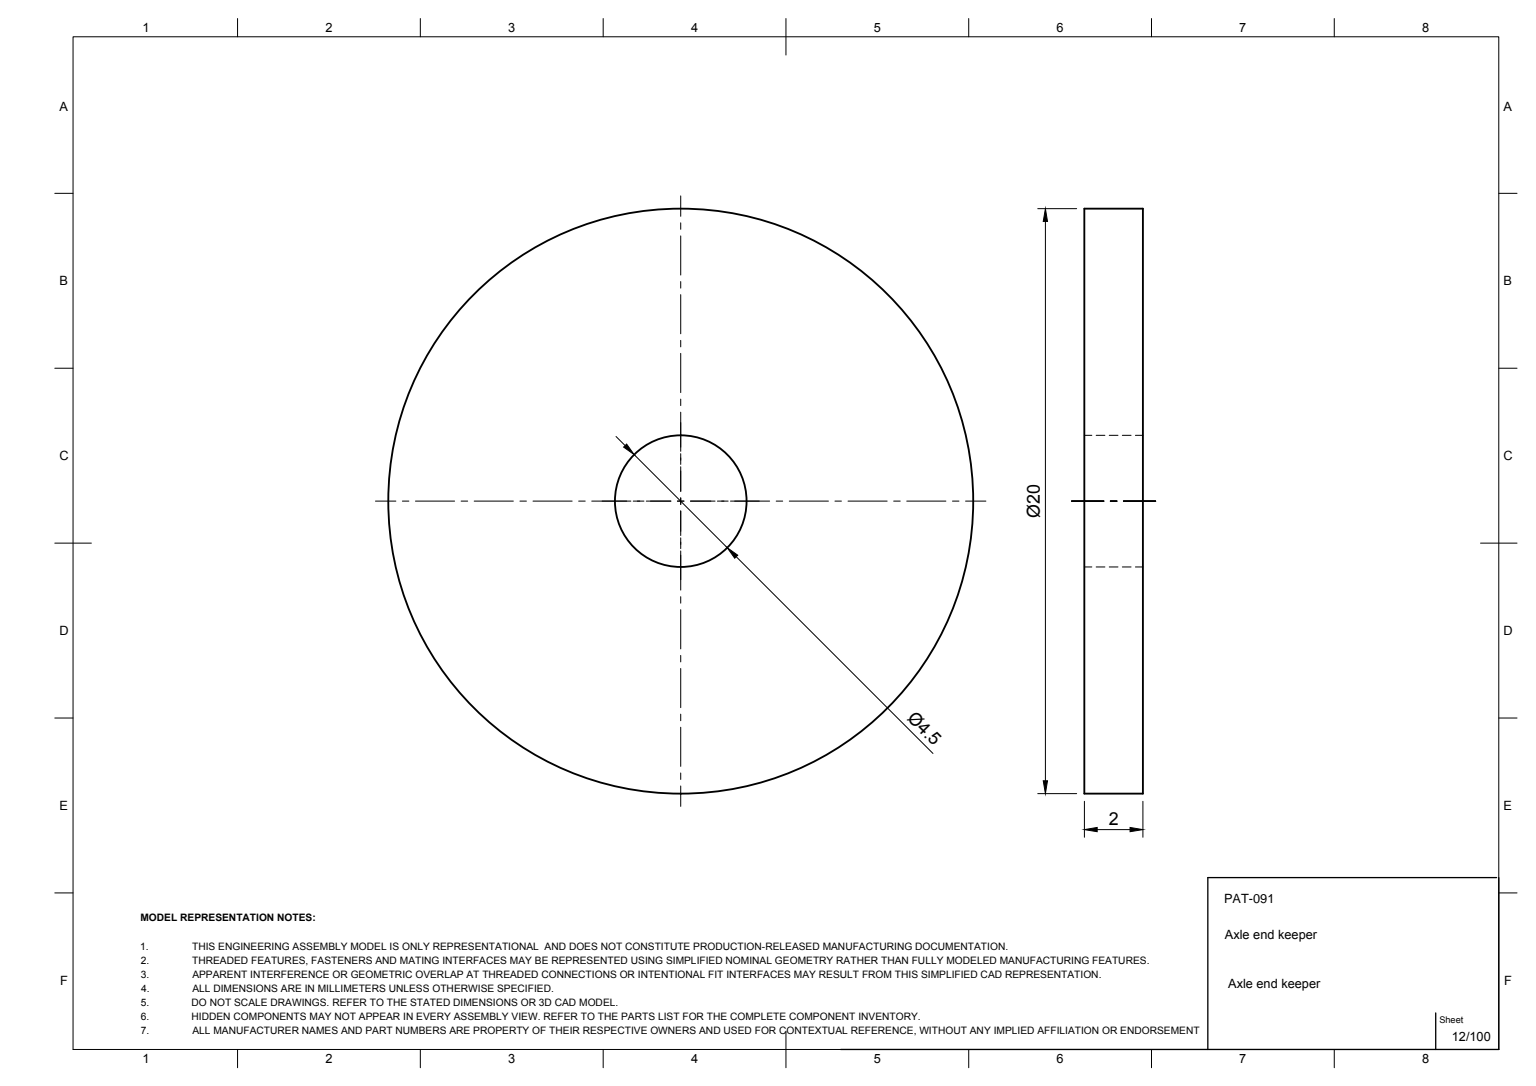
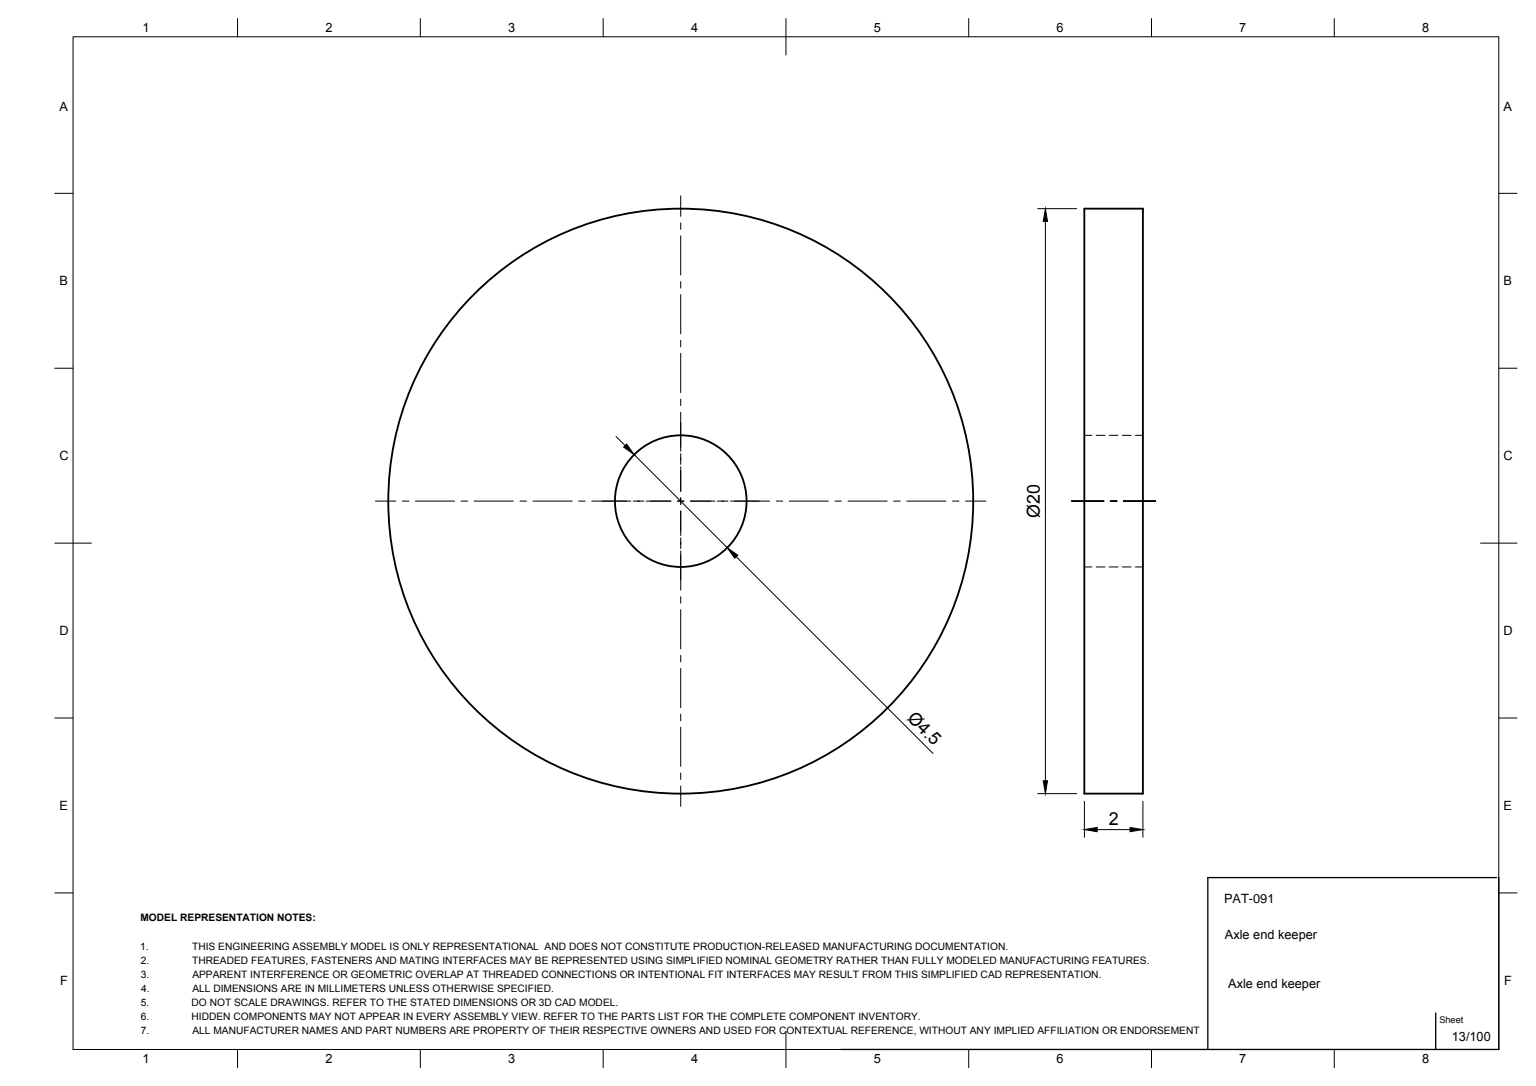
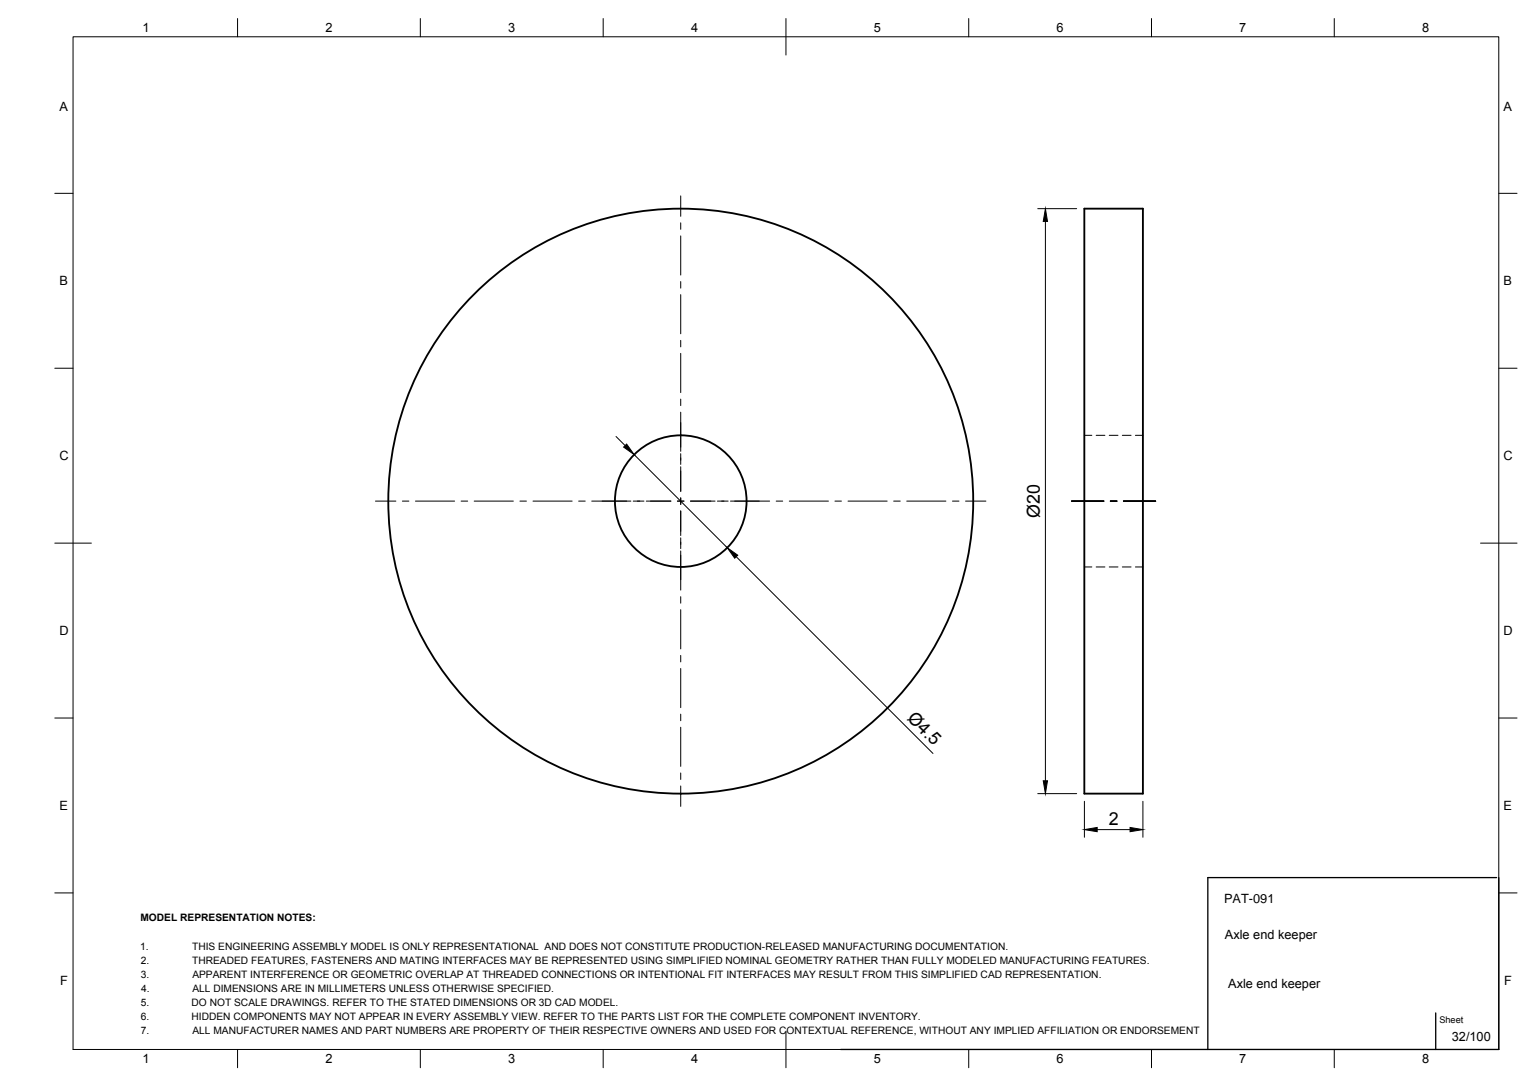
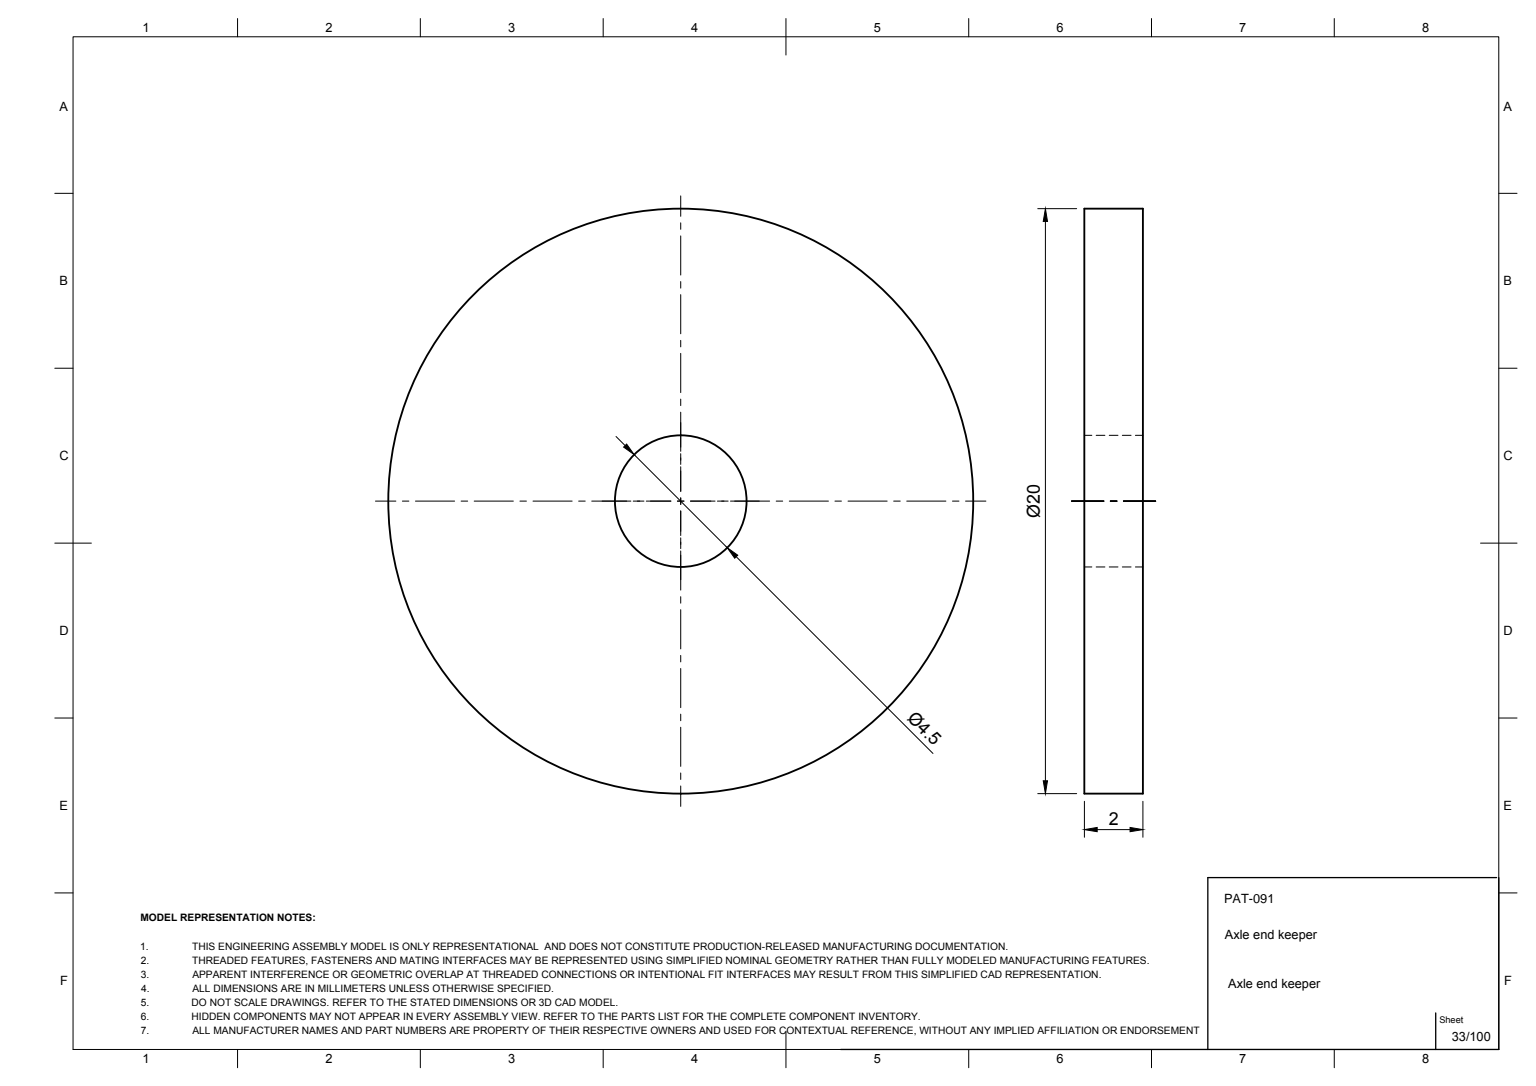
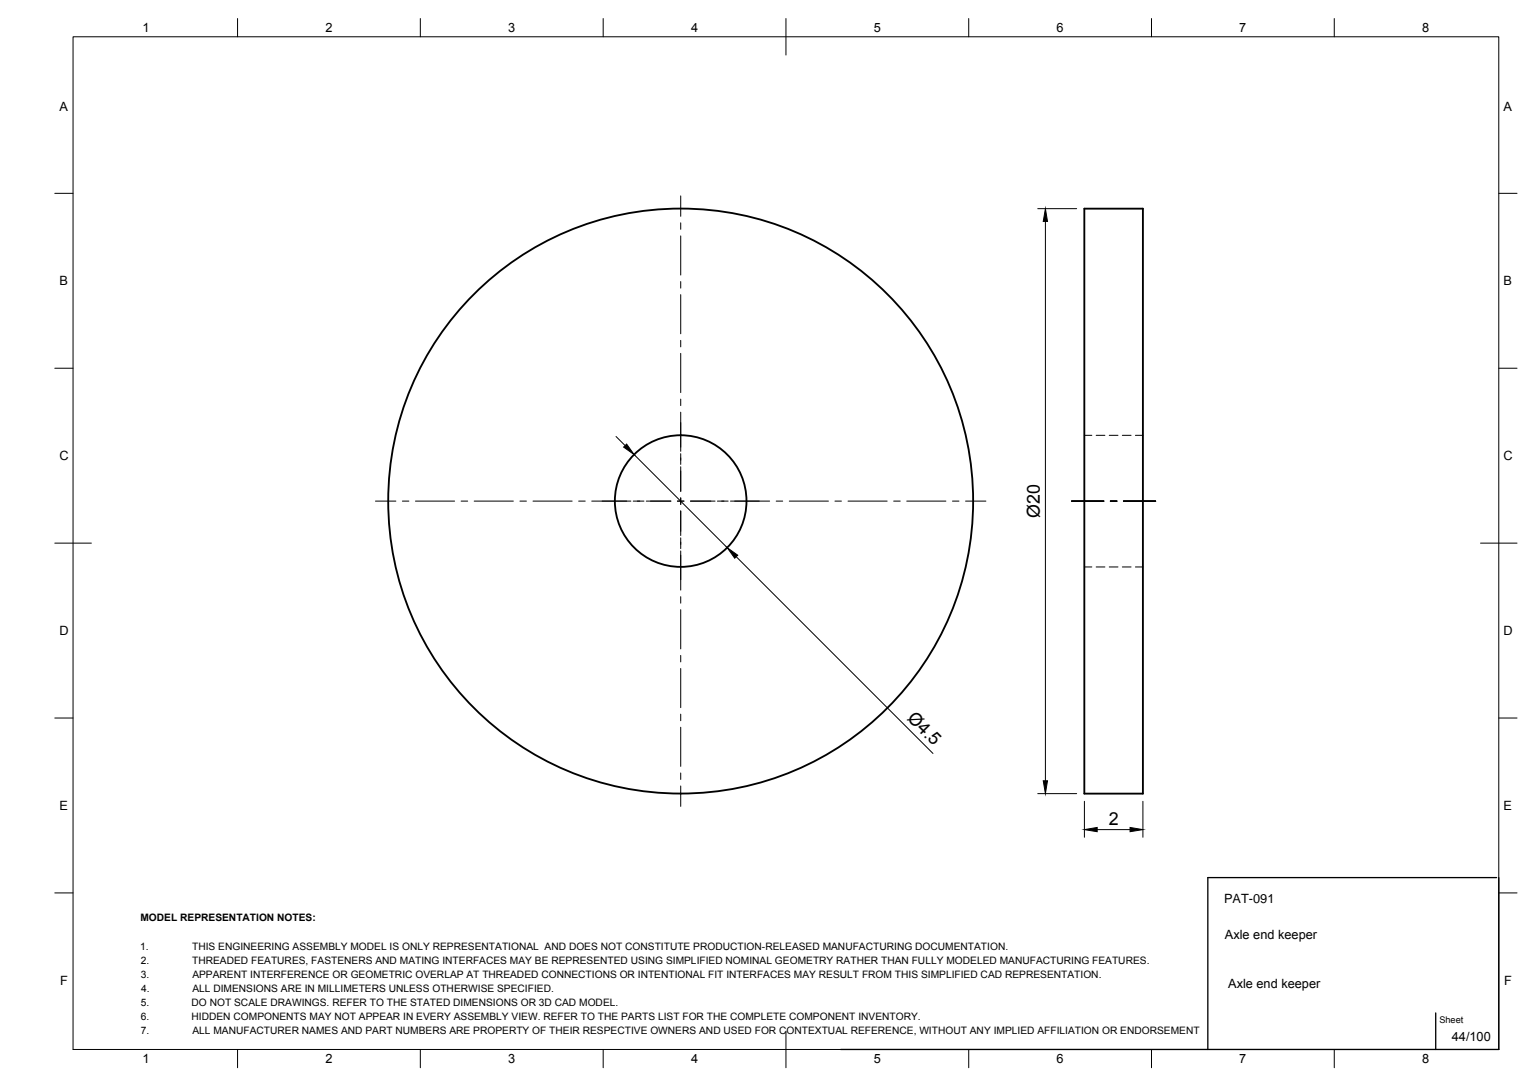
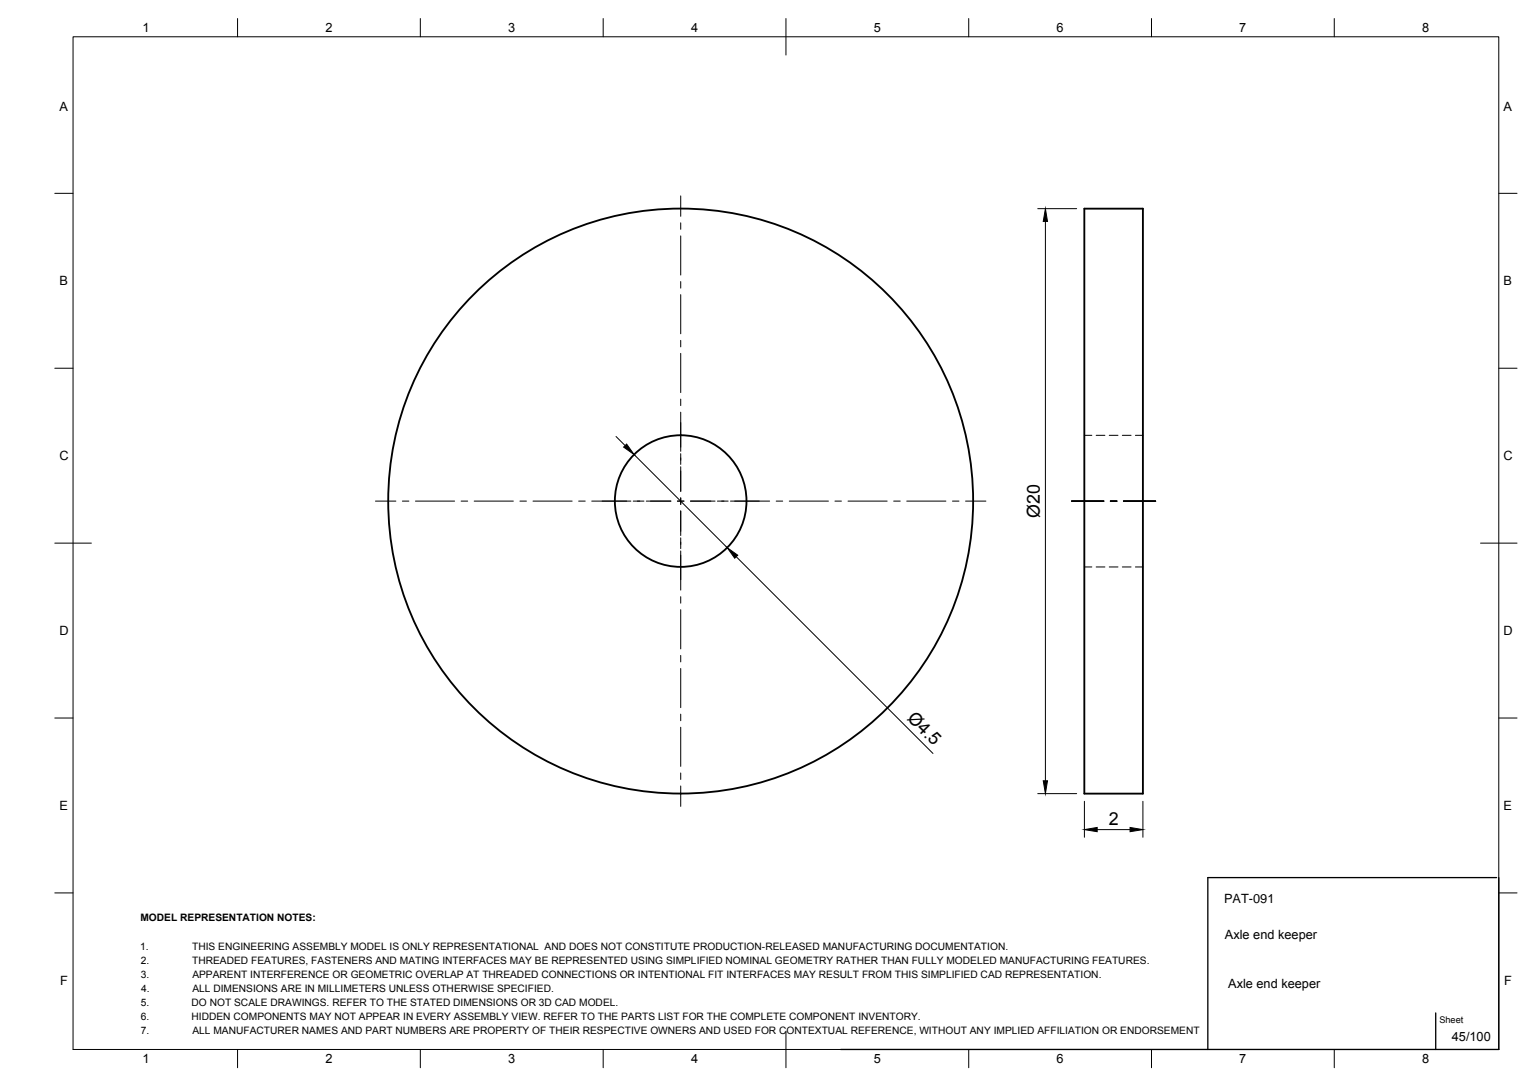
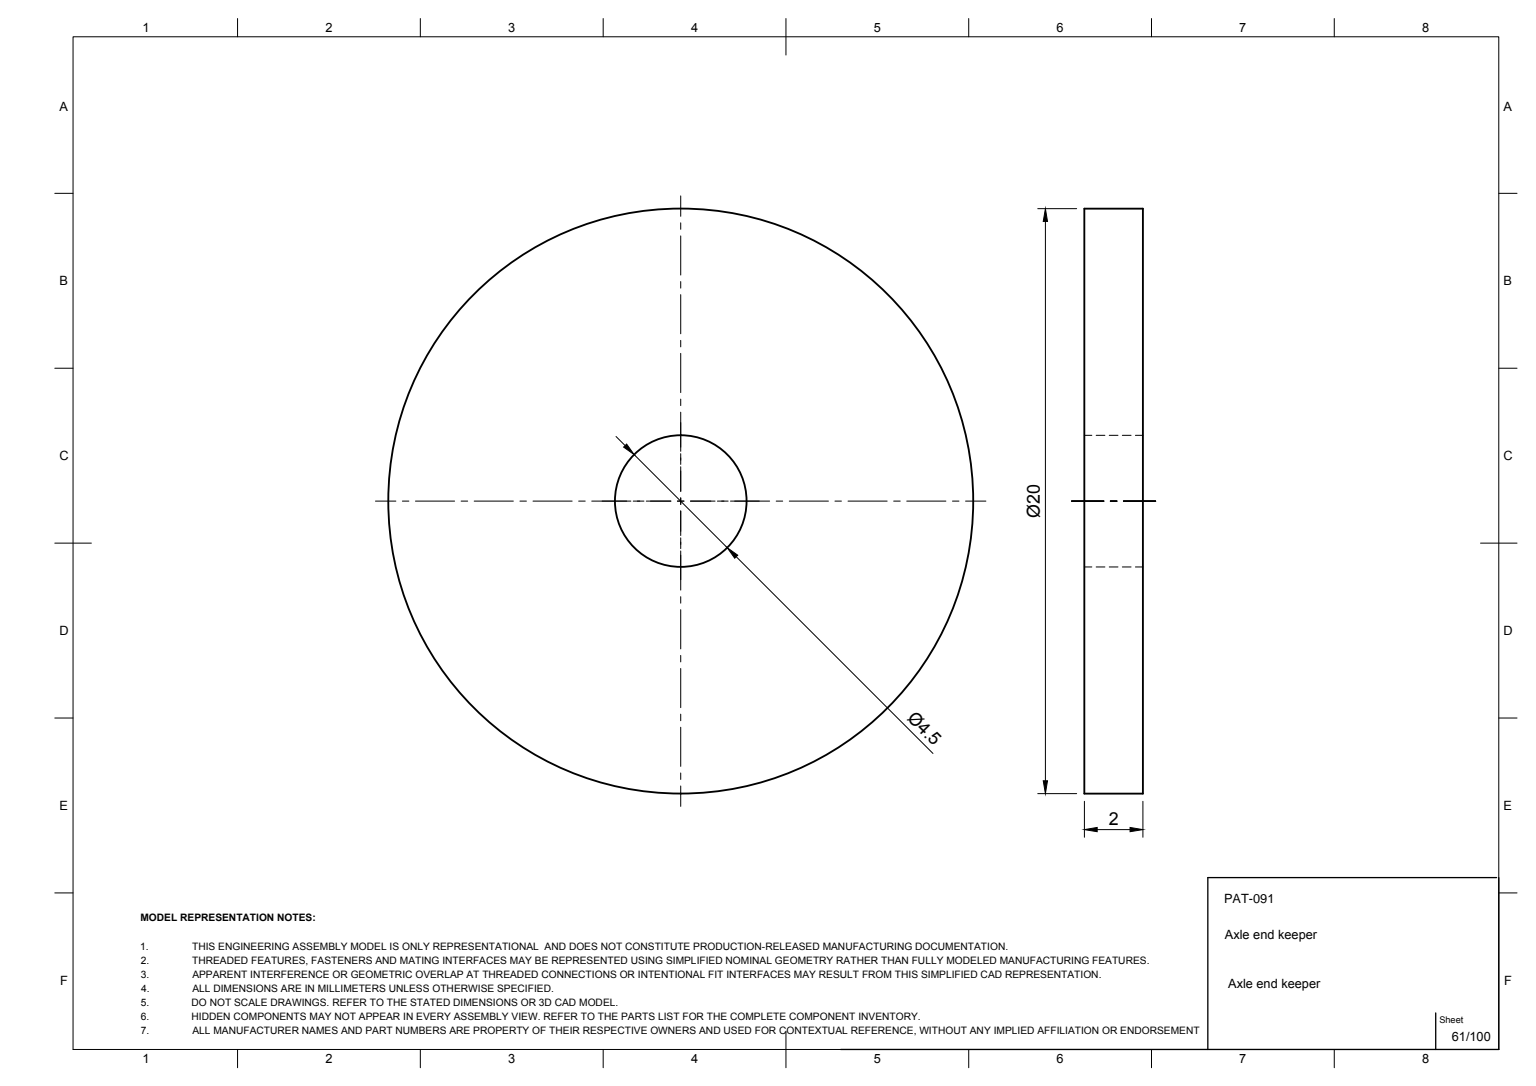
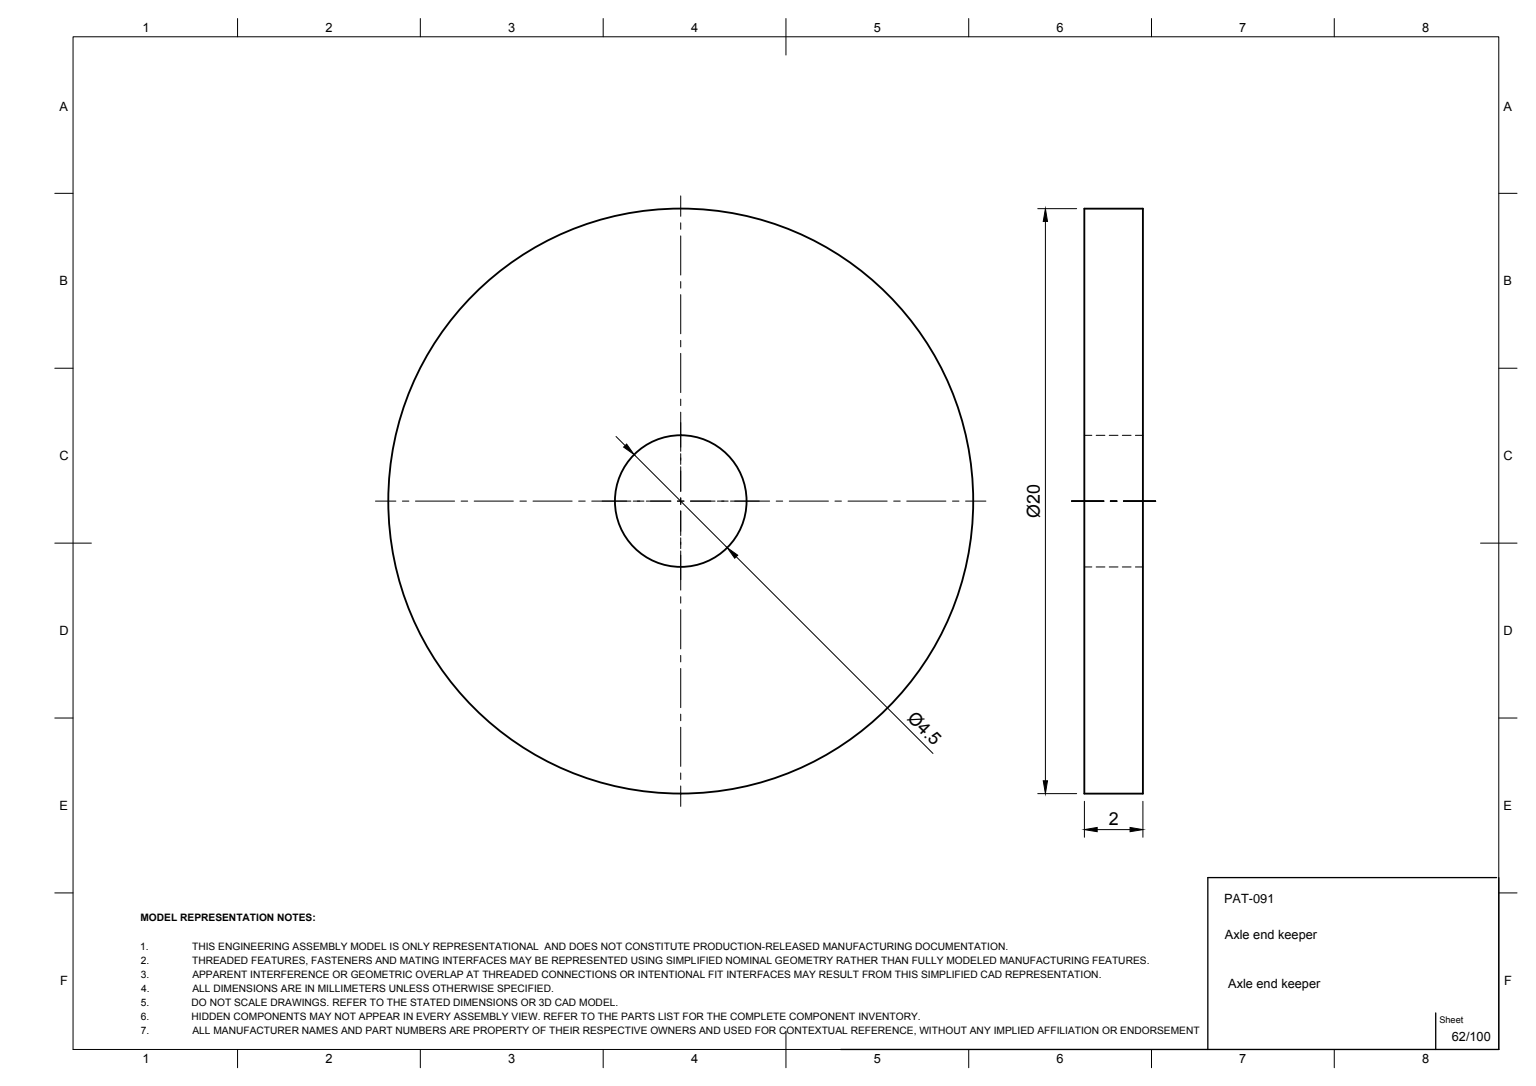
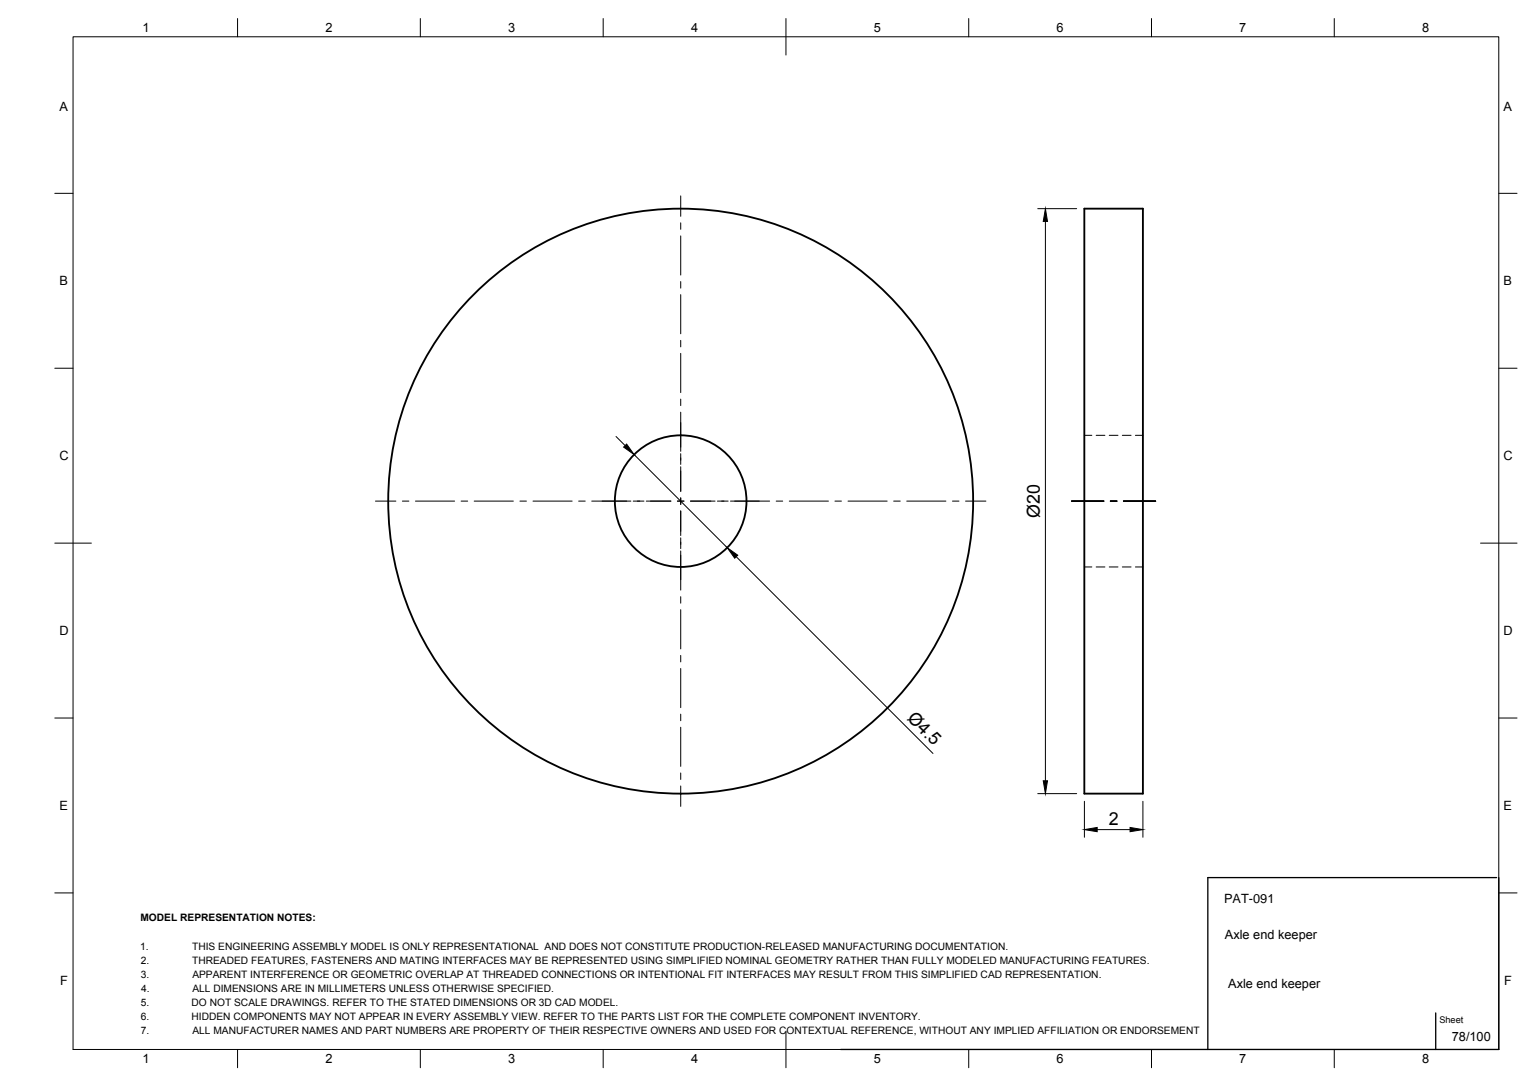
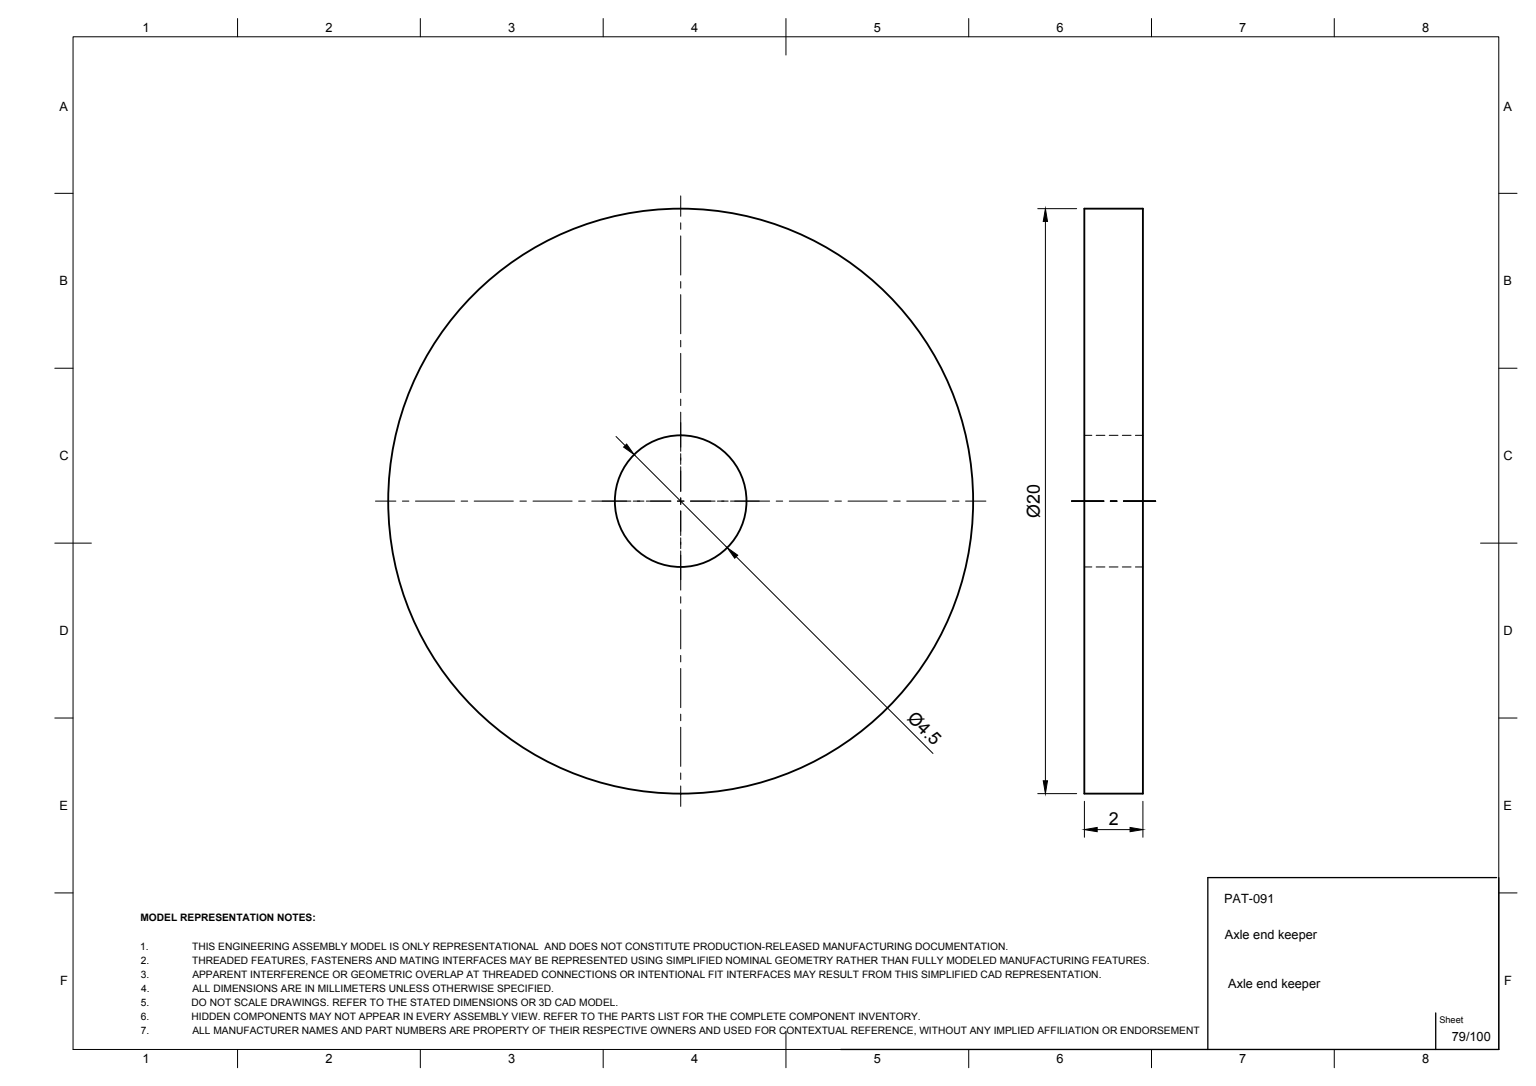
ISO-10303-21;
HEADER;
/* Generated by software containing ST-Developer
 * from STEP Tools, Inc. (www.steptools.com) 
 */

FILE_DESCRIPTION(
/* description */ ('PAT-091'),
/* implementation_level */ '2;1');

FILE_NAME(
/* name */ 'Axle end keeper.step',
/* time_stamp */ '2026-10-27T15:34:44-07:00',
/* author */ (''),
/* organization */ (''),
/* preprocessor_version */ 'ST-DEVELOPER v20.2',
/* originating_system */ 'Autodesk Translation Framework v15.17.0.0',
/* authorisation */ '');

FILE_SCHEMA (('AUTOMOTIVE_DESIGN { 1 0 10303 214 3 1 1 }'));
ENDSEC;

DATA;
#10=MECHANICAL_DESIGN_GEOMETRIC_PRESENTATION_REPRESENTATION('',(#983),#25100);
#763=SHAPE_REPRESENTATION_RELATIONSHIP('SRR','None',#25524,#873);
#873=ADVANCED_BREP_SHAPE_REPRESENTATION('',(#1107),#24994);
#983=STYLED_ITEM('',(#26191),#1107);
#1107=MANIFOLD_SOLID_BREP('Body1',#13260);
#1323=FACE_BOUND('',#3114,.T.);
#1324=FACE_BOUND('',#3116,.T.);
#1698=PLANE('',#14856);
#1699=PLANE('',#14857);
#2185=FACE_OUTER_BOUND('',#3111,.T.);
#2186=FACE_OUTER_BOUND('',#3112,.T.);
#2187=FACE_OUTER_BOUND('',#3113,.T.);
#2188=FACE_OUTER_BOUND('',#3115,.T.);
#3111=EDGE_LOOP('',(#9524,#9525,#9526,#9527));
#3112=EDGE_LOOP('',(#9528,#9529,#9530,#9531));
#3113=EDGE_LOOP('',(#9532));
#3114=EDGE_LOOP('',(#9533));
#3115=EDGE_LOOP('',(#9534));
#3116=EDGE_LOOP('',(#9535));
#4272=LINE('',#21575,#5012);
#4273=LINE('',#21581,#5013);
#5012=VECTOR('',#17150,0.225);
#5013=VECTOR('',#17157,1.);
#5732=CIRCLE('',#14851,0.225);
#5733=CIRCLE('',#14852,0.225);
#5734=CIRCLE('',#14854,1.);
#5735=CIRCLE('',#14855,1.);
#6567=VERTEX_POINT('',#21572);
#6568=VERTEX_POINT('',#21574);
#6569=VERTEX_POINT('',#21578);
#6570=VERTEX_POINT('',#21580);
#7697=EDGE_CURVE('',#6567,#6567,#5732,.T.);
#7698=EDGE_CURVE('',#6567,#6568,#4272,.T.);
#7699=EDGE_CURVE('',#6568,#6568,#5733,.T.);
#7700=EDGE_CURVE('',#6569,#6569,#5734,.T.);
#7701=EDGE_CURVE('',#6569,#6570,#4273,.T.);
#7702=EDGE_CURVE('',#6570,#6570,#5735,.T.);
#9524=ORIENTED_EDGE('',*,*,#7697,.F.);
#9525=ORIENTED_EDGE('',*,*,#7698,.T.);
#9526=ORIENTED_EDGE('',*,*,#7699,.T.);
#9527=ORIENTED_EDGE('',*,*,#7698,.F.);
#9528=ORIENTED_EDGE('',*,*,#7700,.F.);
#9529=ORIENTED_EDGE('',*,*,#7701,.T.);
#9530=ORIENTED_EDGE('',*,*,#7702,.T.);
#9531=ORIENTED_EDGE('',*,*,#7701,.F.);
#9532=ORIENTED_EDGE('',*,*,#7700,.T.);
#9533=ORIENTED_EDGE('',*,*,#7697,.T.);
#9534=ORIENTED_EDGE('',*,*,#7702,.F.);
#9535=ORIENTED_EDGE('',*,*,#7699,.F.);
#12138=CYLINDRICAL_SURFACE('',#14850,0.225);
#12139=CYLINDRICAL_SURFACE('',#14853,1.);
#12552=ADVANCED_FACE('',(#2185),#12138,.F.);
#12553=ADVANCED_FACE('',(#2186),#12139,.T.);
#12554=ADVANCED_FACE('',(#2187,#1323),#1698,.T.);
#12555=ADVANCED_FACE('',(#2188,#1324),#1699,.F.);
#13260=CLOSED_SHELL('',(#12552,#12553,#12554,#12555));
#14849=AXIS2_PLACEMENT_3D('',#21570,#17144,#17145);
#14850=AXIS2_PLACEMENT_3D('',#21571,#17146,#17147);
#14851=AXIS2_PLACEMENT_3D('',#21573,#17148,#17149);
#14852=AXIS2_PLACEMENT_3D('',#21576,#17151,#17152);
#14853=AXIS2_PLACEMENT_3D('',#21577,#17153,#17154);
#14854=AXIS2_PLACEMENT_3D('',#21579,#17155,#17156);
#14855=AXIS2_PLACEMENT_3D('',#21582,#17158,#17159);
#14856=AXIS2_PLACEMENT_3D('',#21583,#17160,#17161);
#14857=AXIS2_PLACEMENT_3D('',#21584,#17162,#17163);
#17144=DIRECTION('axis',(0.,0.,1.));
#17145=DIRECTION('refdir',(1.,0.,0.));
#17146=DIRECTION('center_axis',(0.,1.,0.));
#17147=DIRECTION('ref_axis',(1.,0.,0.));
#17148=DIRECTION('center_axis',(0.,-1.,0.));
#17149=DIRECTION('ref_axis',(1.,0.,0.));
#17150=DIRECTION('',(0.,-1.,0.));
#17151=DIRECTION('center_axis',(0.,-1.,0.));
#17152=DIRECTION('ref_axis',(1.,0.,0.));
#17153=DIRECTION('center_axis',(0.,1.,0.));
#17154=DIRECTION('ref_axis',(1.,0.,0.));
#17155=DIRECTION('center_axis',(0.,1.,0.));
#17156=DIRECTION('ref_axis',(1.,0.,0.));
#17157=DIRECTION('',(0.,-1.,0.));
#17158=DIRECTION('center_axis',(0.,1.,0.));
#17159=DIRECTION('ref_axis',(1.,0.,0.));
#17160=DIRECTION('center_axis',(0.,1.,0.));
#17161=DIRECTION('ref_axis',(1.,0.,0.));
#17162=DIRECTION('center_axis',(0.,1.,0.));
#17163=DIRECTION('ref_axis',(1.,0.,0.));
#21570=CARTESIAN_POINT('',(0.,0.,0.));
#21571=CARTESIAN_POINT('Origin',(0.,-7.7,3.));
#21572=CARTESIAN_POINT('',(-0.225,-7.5,3.));
#21573=CARTESIAN_POINT('Origin',(0.,-7.5,3.));
#21574=CARTESIAN_POINT('',(-0.225,-7.7,3.));
#21575=CARTESIAN_POINT('',(-0.225,-7.7,3.));
#21576=CARTESIAN_POINT('Origin',(0.,-7.7,3.));
#21577=CARTESIAN_POINT('Origin',(0.,-7.7,3.));
#21578=CARTESIAN_POINT('',(-1.,-7.5,3.));
#21579=CARTESIAN_POINT('Origin',(0.,-7.5,3.));
#21580=CARTESIAN_POINT('',(-1.,-7.7,3.));
#21581=CARTESIAN_POINT('',(-1.,-7.7,3.));
#21582=CARTESIAN_POINT('Origin',(0.,-7.7,3.));
#21583=CARTESIAN_POINT('Origin',(0.,-7.5,3.));
#21584=CARTESIAN_POINT('Origin',(0.,-7.7,3.));
#24873=UNCERTAINTY_MEASURE_WITH_UNIT(LENGTH_MEASURE(0.001),#25101,
'DISTANCE_ACCURACY_VALUE',
'Maximum model space distance between geometric entities at asserted c
onnectivities');
#24979=UNCERTAINTY_MEASURE_WITH_UNIT(LENGTH_MEASURE(0.001),#25101,
'DISTANCE_ACCURACY_VALUE',
'Maximum model space distance between geometric entities at asserted c
onnectivities');
#24994=(
GEOMETRIC_REPRESENTATION_CONTEXT(3)
GLOBAL_UNCERTAINTY_ASSIGNED_CONTEXT((#24873))
GLOBAL_UNIT_ASSIGNED_CONTEXT((#25101,#25103,#25104))
REPRESENTATION_CONTEXT('','3D')
);
#25100=(
GEOMETRIC_REPRESENTATION_CONTEXT(3)
GLOBAL_UNCERTAINTY_ASSIGNED_CONTEXT((#24979))
GLOBAL_UNIT_ASSIGNED_CONTEXT((#25101,#25103,#25104))
REPRESENTATION_CONTEXT('','3D')
);
#25101=(
LENGTH_UNIT()
NAMED_UNIT(*)
SI_UNIT(.CENTI.,.METRE.)
);
#25103=(
NAMED_UNIT(*)
PLANE_ANGLE_UNIT()
SI_UNIT($,.RADIAN.)
);
#25104=(
NAMED_UNIT(*)
SI_UNIT($,.STERADIAN.)
SOLID_ANGLE_UNIT()
);
#25119=SHAPE_DEFINITION_REPRESENTATION(#25239,#25524);
#25239=PRODUCT_DEFINITION_SHAPE('',$,#25645);
#25524=SHAPE_REPRESENTATION('',(#14849),#24994);
#25630=PRODUCT_DEFINITION_CONTEXT('part definition',#25992,'design');
#25645=PRODUCT_DEFINITION('Axle end keeper','Axle end keeper',#25765,#25630);
#25765=PRODUCT_DEFINITION_FORMATION('',$,#26008);
#25992=APPLICATION_CONTEXT(
'Core Data for Automotive Mechanical Design Process');
#25993=PRODUCT_CONTEXT('part definition',#25992,'mechanical');
#26008=PRODUCT('Axle end keeper','Axle end keeper','Axle end keeper',(#25993));
#26185=COLOUR_RGB('Grey',0.48,0.52,0.57);
#26186=FILL_AREA_STYLE_COLOUR('',#26185);
#26187=FILL_AREA_STYLE('',(#26186));
#26188=SURFACE_STYLE_FILL_AREA(#26187);
#26189=SURFACE_SIDE_STYLE('',(#26188));
#26190=SURFACE_STYLE_USAGE(.BOTH.,#26189);
#26191=PRESENTATION_STYLE_ASSIGNMENT((#26190));
ENDSEC;
END-ISO-10303-21;
